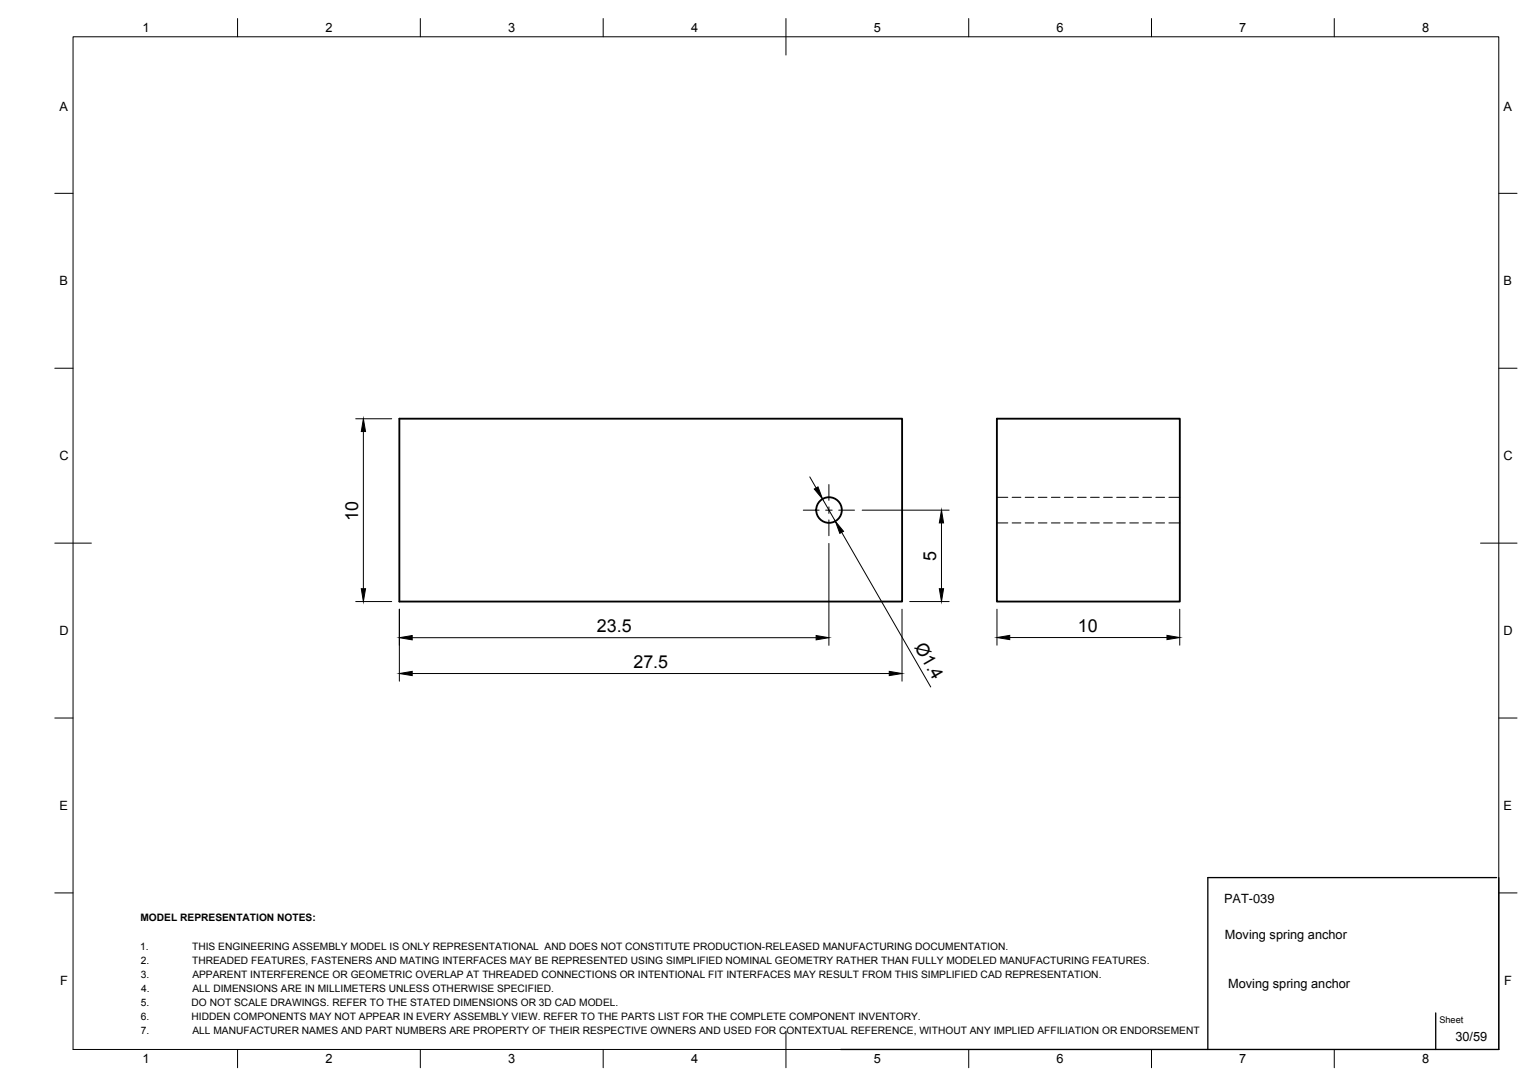
ISO-10303-21;
HEADER;
/* Generated by software containing ST-Developer
 * from STEP Tools, Inc. (www.steptools.com) 
 */

FILE_DESCRIPTION(
/* description */ ('Four-bar parallelogram arm'),
/* implementation_level */ '2;1');

FILE_NAME(
/* name */ 'Moving spring anchor.step',
/* time_stamp */ '2026-10-28T03:24:55-07:00',
/* author */ (''),
/* organization */ (''),
/* preprocessor_version */ 'ST-DEVELOPER v20.2',
/* originating_system */ 'Autodesk Translation Framework v15.17.0.0',
/* authorisation */ '');

FILE_SCHEMA (('AUTOMOTIVE_DESIGN { 1 0 10303 214 3 1 1 }'));
ENDSEC;

DATA;
#10=MECHANICAL_DESIGN_GEOMETRIC_PRESENTATION_REPRESENTATION('',(#646),#14512);
#546=SHAPE_REPRESENTATION_RELATIONSHIP('SRR','None',#14768,#596);
#596=ADVANCED_BREP_SHAPE_REPRESENTATION('',(#703),#14483);
#646=STYLED_ITEM('',(#15087),#703);
#703=MANIFOLD_SOLID_BREP('Body1',#7351);
#871=FACE_BOUND('',#1956,.T.);
#872=FACE_BOUND('',#1959,.T.);
#1105=PLANE('',#8356);
#1106=PLANE('',#8357);
#1107=PLANE('',#8358);
#1108=PLANE('',#8359);
#1109=PLANE('',#8360);
#1110=PLANE('',#8361);
#1397=FACE_OUTER_BOUND('',#1953,.T.);
#1398=FACE_OUTER_BOUND('',#1954,.T.);
#1399=FACE_OUTER_BOUND('',#1955,.T.);
#1400=FACE_OUTER_BOUND('',#1957,.T.);
#1401=FACE_OUTER_BOUND('',#1958,.T.);
#1402=FACE_OUTER_BOUND('',#1960,.T.);
#1403=FACE_OUTER_BOUND('',#1961,.T.);
#1953=EDGE_LOOP('',(#5802,#5803,#5804,#5805));
#1954=EDGE_LOOP('',(#5806,#5807,#5808,#5809));
#1955=EDGE_LOOP('',(#5810,#5811,#5812,#5813));
#1956=EDGE_LOOP('',(#5814));
#1957=EDGE_LOOP('',(#5815,#5816,#5817,#5818));
#1958=EDGE_LOOP('',(#5819,#5820,#5821,#5822));
#1959=EDGE_LOOP('',(#5823));
#1960=EDGE_LOOP('',(#5824,#5825,#5826,#5827));
#1961=EDGE_LOOP('',(#5828,#5829,#5830,#5831));
#2521=LINE('',#12934,#2915);
#2522=LINE('',#12939,#2916);
#2523=LINE('',#12941,#2917);
#2524=LINE('',#12943,#2918);
#2525=LINE('',#12944,#2919);
#2526=LINE('',#12947,#2920);
#2527=LINE('',#12949,#2921);
#2528=LINE('',#12950,#2922);
#2529=LINE('',#12953,#2923);
#2530=LINE('',#12955,#2924);
#2531=LINE('',#12956,#2925);
#2532=LINE('',#12958,#2926);
#2533=LINE('',#12959,#2927);
#2915=VECTOR('',#10013,0.0700000000000003);
#2916=VECTOR('',#10018,1.);
#2917=VECTOR('',#10019,1.);
#2918=VECTOR('',#10020,1.);
#2919=VECTOR('',#10021,1.);
#2920=VECTOR('',#10024,1.);
#2921=VECTOR('',#10025,1.);
#2922=VECTOR('',#10026,1.);
#2923=VECTOR('',#10029,1.);
#2924=VECTOR('',#10030,1.);
#2925=VECTOR('',#10031,1.);
#2926=VECTOR('',#10034,1.);
#2927=VECTOR('',#10035,1.);
#3292=CIRCLE('',#8354,0.0700000000000003);
#3293=CIRCLE('',#8355,0.0700000000000003);
#3814=VERTEX_POINT('',#12931);
#3815=VERTEX_POINT('',#12933);
#3816=VERTEX_POINT('',#12937);
#3817=VERTEX_POINT('',#12938);
#3818=VERTEX_POINT('',#12940);
#3819=VERTEX_POINT('',#12942);
#3820=VERTEX_POINT('',#12946);
#3821=VERTEX_POINT('',#12948);
#3822=VERTEX_POINT('',#12952);
#3823=VERTEX_POINT('',#12954);
#4532=EDGE_CURVE('',#3814,#3814,#3292,.T.);
#4533=EDGE_CURVE('',#3814,#3815,#2521,.T.);
#4534=EDGE_CURVE('',#3815,#3815,#3293,.T.);
#4535=EDGE_CURVE('',#3816,#3817,#2522,.T.);
#4536=EDGE_CURVE('',#3817,#3818,#2523,.T.);
#4537=EDGE_CURVE('',#3819,#3818,#2524,.T.);
#4538=EDGE_CURVE('',#3816,#3819,#2525,.T.);
#4539=EDGE_CURVE('',#3820,#3816,#2526,.T.);
#4540=EDGE_CURVE('',#3821,#3819,#2527,.T.);
#4541=EDGE_CURVE('',#3820,#3821,#2528,.T.);
#4542=EDGE_CURVE('',#3822,#3820,#2529,.T.);
#4543=EDGE_CURVE('',#3823,#3821,#2530,.T.);
#4544=EDGE_CURVE('',#3822,#3823,#2531,.T.);
#4545=EDGE_CURVE('',#3817,#3822,#2532,.T.);
#4546=EDGE_CURVE('',#3818,#3823,#2533,.T.);
#5802=ORIENTED_EDGE('',*,*,#4532,.F.);
#5803=ORIENTED_EDGE('',*,*,#4533,.T.);
#5804=ORIENTED_EDGE('',*,*,#4534,.F.);
#5805=ORIENTED_EDGE('',*,*,#4533,.F.);
#5806=ORIENTED_EDGE('',*,*,#4535,.T.);
#5807=ORIENTED_EDGE('',*,*,#4536,.T.);
#5808=ORIENTED_EDGE('',*,*,#4537,.F.);
#5809=ORIENTED_EDGE('',*,*,#4538,.F.);
#5810=ORIENTED_EDGE('',*,*,#4539,.T.);
#5811=ORIENTED_EDGE('',*,*,#4538,.T.);
#5812=ORIENTED_EDGE('',*,*,#4540,.F.);
#5813=ORIENTED_EDGE('',*,*,#4541,.F.);
#5814=ORIENTED_EDGE('',*,*,#4534,.T.);
#5815=ORIENTED_EDGE('',*,*,#4542,.T.);
#5816=ORIENTED_EDGE('',*,*,#4541,.T.);
#5817=ORIENTED_EDGE('',*,*,#4543,.F.);
#5818=ORIENTED_EDGE('',*,*,#4544,.F.);
#5819=ORIENTED_EDGE('',*,*,#4545,.T.);
#5820=ORIENTED_EDGE('',*,*,#4544,.T.);
#5821=ORIENTED_EDGE('',*,*,#4546,.F.);
#5822=ORIENTED_EDGE('',*,*,#4536,.F.);
#5823=ORIENTED_EDGE('',*,*,#4532,.T.);
#5824=ORIENTED_EDGE('',*,*,#4546,.T.);
#5825=ORIENTED_EDGE('',*,*,#4543,.T.);
#5826=ORIENTED_EDGE('',*,*,#4540,.T.);
#5827=ORIENTED_EDGE('',*,*,#4537,.T.);
#5828=ORIENTED_EDGE('',*,*,#4545,.F.);
#5829=ORIENTED_EDGE('',*,*,#4535,.F.);
#5830=ORIENTED_EDGE('',*,*,#4539,.F.);
#5831=ORIENTED_EDGE('',*,*,#4542,.F.);
#6807=CYLINDRICAL_SURFACE('',#8353,0.0700000000000003);
#7102=ADVANCED_FACE('',(#1397),#6807,.F.);
#7103=ADVANCED_FACE('',(#1398),#1105,.T.);
#7104=ADVANCED_FACE('',(#1399,#871),#1106,.T.);
#7105=ADVANCED_FACE('',(#1400),#1107,.T.);
#7106=ADVANCED_FACE('',(#1401,#872),#1108,.T.);
#7107=ADVANCED_FACE('',(#1402),#1109,.T.);
#7108=ADVANCED_FACE('',(#1403),#1110,.F.);
#7351=CLOSED_SHELL('',(#7102,#7103,#7104,#7105,#7106,#7107,#7108));
#8352=AXIS2_PLACEMENT_3D('',#12929,#10007,#10008);
#8353=AXIS2_PLACEMENT_3D('',#12930,#10009,#10010);
#8354=AXIS2_PLACEMENT_3D('',#12932,#10011,#10012);
#8355=AXIS2_PLACEMENT_3D('',#12935,#10014,#10015);
#8356=AXIS2_PLACEMENT_3D('',#12936,#10016,#10017);
#8357=AXIS2_PLACEMENT_3D('',#12945,#10022,#10023);
#8358=AXIS2_PLACEMENT_3D('',#12951,#10027,#10028);
#8359=AXIS2_PLACEMENT_3D('',#12957,#10032,#10033);
#8360=AXIS2_PLACEMENT_3D('',#12960,#10036,#10037);
#8361=AXIS2_PLACEMENT_3D('',#12961,#10038,#10039);
#10007=DIRECTION('axis',(0.,0.,1.));
#10008=DIRECTION('refdir',(1.,0.,0.));
#10009=DIRECTION('center_axis',(1.,0.,0.));
#10010=DIRECTION('ref_axis',(0.,0.,-1.));
#10011=DIRECTION('center_axis',(1.,0.,0.));
#10012=DIRECTION('ref_axis',(0.,0.,-1.));
#10013=DIRECTION('',(1.,0.,0.));
#10014=DIRECTION('center_axis',(-1.,0.,0.));
#10015=DIRECTION('ref_axis',(0.,0.,-1.));
#10016=DIRECTION('center_axis',(0.,1.,0.));
#10017=DIRECTION('ref_axis',(-1.,0.,0.));
#10018=DIRECTION('',(-1.,0.,0.));
#10019=DIRECTION('',(0.,0.,1.));
#10020=DIRECTION('',(-1.,0.,0.));
#10021=DIRECTION('',(0.,0.,1.));
#10022=DIRECTION('center_axis',(1.,0.,0.));
#10023=DIRECTION('ref_axis',(0.,1.,0.));
#10024=DIRECTION('',(0.,1.,0.));
#10025=DIRECTION('',(0.,1.,0.));
#10026=DIRECTION('',(0.,0.,1.));
#10027=DIRECTION('center_axis',(0.,-1.,0.));
#10028=DIRECTION('ref_axis',(1.,0.,0.));
#10029=DIRECTION('',(1.,0.,0.));
#10030=DIRECTION('',(1.,0.,0.));
#10031=DIRECTION('',(0.,0.,1.));
#10032=DIRECTION('center_axis',(-1.,0.,0.));
#10033=DIRECTION('ref_axis',(0.,-1.,0.));
#10034=DIRECTION('',(0.,-1.,0.));
#10035=DIRECTION('',(0.,-1.,0.));
#10036=DIRECTION('center_axis',(0.,0.,1.));
#10037=DIRECTION('ref_axis',(1.,0.,0.));
#10038=DIRECTION('center_axis',(0.,0.,1.));
#10039=DIRECTION('ref_axis',(1.,0.,0.));
#12929=CARTESIAN_POINT('',(0.,0.,0.));
#12930=CARTESIAN_POINT('Origin',(3.4,-3.4,8.));
#12931=CARTESIAN_POINT('',(3.5,-3.4,8.07));
#12932=CARTESIAN_POINT('Origin',(3.5,-3.4,8.));
#12933=CARTESIAN_POINT('',(4.5,-3.4,8.07));
#12934=CARTESIAN_POINT('',(3.4,-3.4,8.07));
#12935=CARTESIAN_POINT('Origin',(4.5,-3.4,8.));
#12936=CARTESIAN_POINT('Origin',(4.5,-1.05,7.5));
#12937=CARTESIAN_POINT('',(4.5,-1.05,7.5));
#12938=CARTESIAN_POINT('',(3.5,-1.05,7.5));
#12939=CARTESIAN_POINT('',(4.5,-1.05,7.5));
#12940=CARTESIAN_POINT('',(3.5,-1.05,8.5));
#12941=CARTESIAN_POINT('',(3.5,-1.05,7.5));
#12942=CARTESIAN_POINT('',(4.5,-1.05,8.5));
#12943=CARTESIAN_POINT('',(4.5,-1.05,8.5));
#12944=CARTESIAN_POINT('',(4.5,-1.05,7.5));
#12945=CARTESIAN_POINT('Origin',(4.5,-3.8,7.5));
#12946=CARTESIAN_POINT('',(4.5,-3.8,7.5));
#12947=CARTESIAN_POINT('',(4.5,-3.8,7.5));
#12948=CARTESIAN_POINT('',(4.5,-3.8,8.5));
#12949=CARTESIAN_POINT('',(4.5,-3.8,8.5));
#12950=CARTESIAN_POINT('',(4.5,-3.8,7.5));
#12951=CARTESIAN_POINT('Origin',(3.5,-3.8,7.5));
#12952=CARTESIAN_POINT('',(3.5,-3.8,7.5));
#12953=CARTESIAN_POINT('',(3.5,-3.8,7.5));
#12954=CARTESIAN_POINT('',(3.5,-3.8,8.5));
#12955=CARTESIAN_POINT('',(3.5,-3.8,8.5));
#12956=CARTESIAN_POINT('',(3.5,-3.8,7.5));
#12957=CARTESIAN_POINT('Origin',(3.5,-1.05,7.5));
#12958=CARTESIAN_POINT('',(3.5,-1.05,7.5));
#12959=CARTESIAN_POINT('',(3.5,-1.05,8.5));
#12960=CARTESIAN_POINT('Origin',(4.,-2.425,8.5));
#12961=CARTESIAN_POINT('Origin',(4.,-2.425,7.5));
#14426=UNCERTAINTY_MEASURE_WITH_UNIT(LENGTH_MEASURE(0.001),#14513,
'DISTANCE_ACCURACY_VALUE',
'Maximum model space distance between geometric entities at asserted c
onnectivities');
#14455=UNCERTAINTY_MEASURE_WITH_UNIT(LENGTH_MEASURE(0.001),#14513,
'DISTANCE_ACCURACY_VALUE',
'Maximum model space distance between geometric entities at asserted c
onnectivities');
#14483=(
GEOMETRIC_REPRESENTATION_CONTEXT(3)
GLOBAL_UNCERTAINTY_ASSIGNED_CONTEXT((#14426))
GLOBAL_UNIT_ASSIGNED_CONTEXT((#14513,#14515,#14516))
REPRESENTATION_CONTEXT('','3D')
);
#14512=(
GEOMETRIC_REPRESENTATION_CONTEXT(3)
GLOBAL_UNCERTAINTY_ASSIGNED_CONTEXT((#14455))
GLOBAL_UNIT_ASSIGNED_CONTEXT((#14513,#14515,#14516))
REPRESENTATION_CONTEXT('','3D')
);
#14513=(
LENGTH_UNIT()
NAMED_UNIT(*)
SI_UNIT(.CENTI.,.METRE.)
);
#14515=(
NAMED_UNIT(*)
PLANE_ANGLE_UNIT()
SI_UNIT($,.RADIAN.)
);
#14516=(
NAMED_UNIT(*)
SI_UNIT($,.STERADIAN.)
SOLID_ANGLE_UNIT()
);
#14544=SHAPE_DEFINITION_REPRESENTATION(#14600,#14768);
#14600=PRODUCT_DEFINITION_SHAPE('',$,#14825);
#14768=SHAPE_REPRESENTATION('',(#8352),#14483);
#14797=PRODUCT_DEFINITION_CONTEXT('part definition',#14967,'design');
#14825=PRODUCT_DEFINITION('Moving spring anchor','Moving spring anchor',
#14881,#14797);
#14881=PRODUCT_DEFINITION_FORMATION('',$,#14996);
#14967=APPLICATION_CONTEXT(
'Core Data for Automotive Mechanical Design Process');
#14968=PRODUCT_CONTEXT('part definition',#14967,'mechanical');
#14996=PRODUCT('Moving spring anchor','Moving spring anchor',
'Moving spring anchor',(#14968));
#15081=COLOUR_RGB('Grey',0.48,0.52,0.57);
#15082=FILL_AREA_STYLE_COLOUR('',#15081);
#15083=FILL_AREA_STYLE('',(#15082));
#15084=SURFACE_STYLE_FILL_AREA(#15083);
#15085=SURFACE_SIDE_STYLE('',(#15084));
#15086=SURFACE_STYLE_USAGE(.BOTH.,#15085);
#15087=PRESENTATION_STYLE_ASSIGNMENT((#15086));
ENDSEC;
END-ISO-10303-21;
